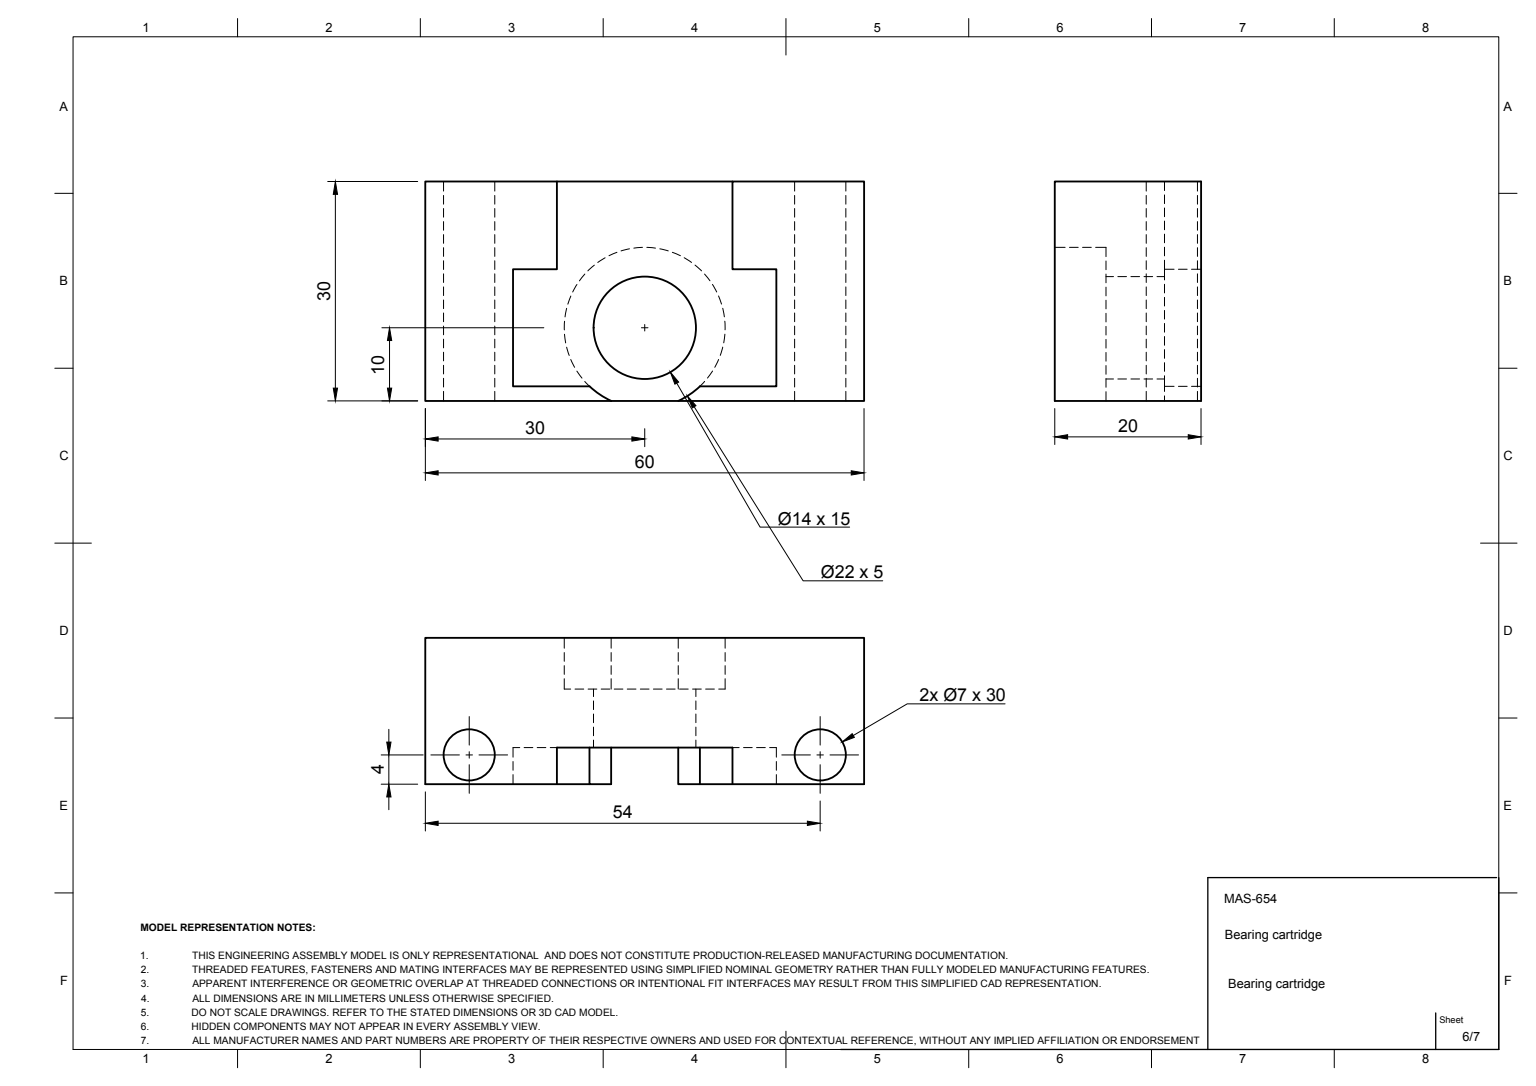
ISO-10303-21;
HEADER;
/* Generated by software containing ST-Developer
 * from STEP Tools, Inc. (www.steptools.com) 
 */

FILE_DESCRIPTION(
/* description */ ('Independent four-jaw lathe chuck,200mm body,40mm bore,36\X2\2013\X0\7
6mm nominal opposed jaw opening. Four shared machined T-jaws and model
ed partial M12x1.75 feed screws, native independent screw/slider links
, removable bolted bronze-bearing cartridges, fully captured ring/wash
er/head thrust stacks and registered bolted backplate. Custom spindle 
interface; no compatibility, speed, grip force or safety rating assign
ed.'),
/* implementation_level */ '2;1');

FILE_NAME(
/* name */ 'Bearing cartridge.step',
/* time_stamp */ '2026-11-09T20:24:54-08:00',
/* author */ (''),
/* organization */ (''),
/* preprocessor_version */ 'ST-DEVELOPER v20.2',
/* originating_system */ 'Autodesk Translation Framework v15.17.0.0',
/* authorisation */ '');

FILE_SCHEMA (('AUTOMOTIVE_DESIGN { 1 0 10303 214 3 1 1 }'));
ENDSEC;

DATA;
#10=MECHANICAL_DESIGN_GEOMETRIC_PRESENTATION_REPRESENTATION('',(#239),#69491);
#217=SHAPE_REPRESENTATION_RELATIONSHIP('SRR','None',#69574,#228);
#228=ADVANCED_BREP_SHAPE_REPRESENTATION('',(#250),#69483);
#239=STYLED_ITEM('',(#69638),#250);
#250=MANIFOLD_SOLID_BREP('Body1',#14734);
#345=FACE_BOUND('',#1827,.T.);
#346=FACE_BOUND('',#1832,.T.);
#347=FACE_BOUND('',#1835,.T.);
#348=FACE_BOUND('',#1836,.T.);
#349=FACE_BOUND('',#1849,.T.);
#350=FACE_BOUND('',#1850,.T.);
#462=PLANE('',#15459);
#463=PLANE('',#15461);
#464=PLANE('',#15462);
#465=PLANE('',#15463);
#466=PLANE('',#15464);
#467=PLANE('',#15469);
#468=PLANE('',#15471);
#469=PLANE('',#15472);
#470=PLANE('',#15473);
#471=PLANE('',#15474);
#472=PLANE('',#15475);
#473=PLANE('',#15476);
#474=PLANE('',#15477);
#475=PLANE('',#15478);
#476=PLANE('',#15479);
#477=PLANE('',#15480);
#478=PLANE('',#15481);
#994=FACE_OUTER_BOUND('',#1822,.T.);
#995=FACE_OUTER_BOUND('',#1823,.T.);
#996=FACE_OUTER_BOUND('',#1824,.T.);
#997=FACE_OUTER_BOUND('',#1825,.T.);
#998=FACE_OUTER_BOUND('',#1826,.T.);
#999=FACE_OUTER_BOUND('',#1828,.T.);
#1000=FACE_OUTER_BOUND('',#1829,.T.);
#1001=FACE_OUTER_BOUND('',#1830,.T.);
#1002=FACE_OUTER_BOUND('',#1831,.T.);
#1003=FACE_OUTER_BOUND('',#1833,.T.);
#1004=FACE_OUTER_BOUND('',#1834,.T.);
#1005=FACE_OUTER_BOUND('',#1837,.T.);
#1006=FACE_OUTER_BOUND('',#1838,.T.);
#1007=FACE_OUTER_BOUND('',#1839,.T.);
#1008=FACE_OUTER_BOUND('',#1840,.T.);
#1009=FACE_OUTER_BOUND('',#1841,.T.);
#1010=FACE_OUTER_BOUND('',#1842,.T.);
#1011=FACE_OUTER_BOUND('',#1843,.T.);
#1012=FACE_OUTER_BOUND('',#1844,.T.);
#1013=FACE_OUTER_BOUND('',#1845,.T.);
#1014=FACE_OUTER_BOUND('',#1846,.T.);
#1015=FACE_OUTER_BOUND('',#1847,.T.);
#1016=FACE_OUTER_BOUND('',#1848,.T.);
#1822=EDGE_LOOP('',(#11663,#11664,#11665,#11666));
#1823=EDGE_LOOP('',(#11667,#11668,#11669,#11670));
#1824=EDGE_LOOP('',(#11671,#11672,#11673,#11674));
#1825=EDGE_LOOP('',(#11675,#11676,#11677,#11678));
#1826=EDGE_LOOP('',(#11679,#11680,#11681,#11682,#11683,#11684,#11685,#11686,
#11687,#11688,#11689,#11690));
#1827=EDGE_LOOP('',(#11691));
#1828=EDGE_LOOP('',(#11692,#11693,#11694,#11695,#11696,#11697,#11698,#11699));
#1829=EDGE_LOOP('',(#11700,#11701,#11702,#11703,#11704,#11705,#11706,#11707));
#1830=EDGE_LOOP('',(#11708,#11709,#11710,#11711));
#1831=EDGE_LOOP('',(#11712,#11713));
#1832=EDGE_LOOP('',(#11714));
#1833=EDGE_LOOP('',(#11715,#11716,#11717,#11718));
#1834=EDGE_LOOP('',(#11719,#11720,#11721,#11722,#11723,#11724,#11725,#11726,
#11727,#11728,#11729,#11730));
#1835=EDGE_LOOP('',(#11731));
#1836=EDGE_LOOP('',(#11732));
#1837=EDGE_LOOP('',(#11733,#11734,#11735,#11736));
#1838=EDGE_LOOP('',(#11737,#11738,#11739,#11740));
#1839=EDGE_LOOP('',(#11741,#11742,#11743,#11744));
#1840=EDGE_LOOP('',(#11745,#11746,#11747,#11748));
#1841=EDGE_LOOP('',(#11749,#11750,#11751,#11752));
#1842=EDGE_LOOP('',(#11753,#11754,#11755,#11756));
#1843=EDGE_LOOP('',(#11757,#11758,#11759,#11760));
#1844=EDGE_LOOP('',(#11761,#11762,#11763,#11764));
#1845=EDGE_LOOP('',(#11765,#11766,#11767,#11768));
#1846=EDGE_LOOP('',(#11769,#11770,#11771,#11772,#11773,#11774));
#1847=EDGE_LOOP('',(#11775,#11776,#11777,#11778));
#1848=EDGE_LOOP('',(#11779,#11780,#11781,#11782,#11783,#11784,#11785,#11786));
#1849=EDGE_LOOP('',(#11787));
#1850=EDGE_LOOP('',(#11788));
#2291=CIRCLE('',#15448,3.5);
#2292=CIRCLE('',#15449,3.5);
#2293=CIRCLE('',#15451,3.5);
#2294=CIRCLE('',#15452,3.5);
#2295=CIRCLE('',#15454,11.);
#2296=CIRCLE('',#15455,11.);
#2297=CIRCLE('',#15457,11.);
#2298=CIRCLE('',#15458,11.);
#2299=CIRCLE('',#15460,7.);
#2300=CIRCLE('',#15465,11.);
#2301=CIRCLE('',#15466,7.);
#2302=CIRCLE('',#15468,11.);
#4032=LINE('',#50300,#4880);
#4033=LINE('',#50306,#4881);
#4034=LINE('',#50311,#4882);
#4035=LINE('',#50315,#4883);
#4036=LINE('',#50320,#4884);
#4037=LINE('',#50324,#4885);
#4038=LINE('',#50328,#4886);
#4039=LINE('',#50330,#4887);
#4040=LINE('',#50332,#4888);
#4041=LINE('',#50334,#4889);
#4042=LINE('',#50336,#4890);
#4043=LINE('',#50338,#4891);
#4044=LINE('',#50340,#4892);
#4045=LINE('',#50342,#4893);
#4046=LINE('',#50343,#4894);
#4047=LINE('',#50344,#4895);
#4048=LINE('',#50349,#4896);
#4049=LINE('',#50351,#4897);
#4050=LINE('',#50353,#4898);
#4051=LINE('',#50355,#4899);
#4052=LINE('',#50357,#4900);
#4053=LINE('',#50359,#4901);
#4054=LINE('',#50360,#4902);
#4055=LINE('',#50363,#4903);
#4056=LINE('',#50365,#4904);
#4057=LINE('',#50367,#4905);
#4058=LINE('',#50369,#4906);
#4059=LINE('',#50371,#4907);
#4060=LINE('',#50373,#4908);
#4061=LINE('',#50374,#4909);
#4062=LINE('',#50376,#4910);
#4063=LINE('',#50380,#4911);
#4064=LINE('',#50386,#4912);
#4065=LINE('',#50389,#4913);
#4066=LINE('',#50392,#4914);
#4067=LINE('',#50393,#4915);
#4068=LINE('',#50395,#4916);
#4069=LINE('',#50396,#4917);
#4070=LINE('',#50398,#4918);
#4071=LINE('',#50400,#4919);
#4072=LINE('',#50401,#4920);
#4073=LINE('',#50404,#4921);
#4074=LINE('',#50405,#4922);
#4075=LINE('',#50407,#4923);
#4076=LINE('',#50410,#4924);
#4077=LINE('',#50412,#4925);
#4078=LINE('',#50415,#4926);
#4079=LINE('',#50416,#4927);
#4080=LINE('',#50419,#4928);
#4081=LINE('',#50420,#4929);
#4082=LINE('',#50422,#4930);
#4880=VECTOR('',#17538,3.5);
#4881=VECTOR('',#17545,3.5);
#4882=VECTOR('',#17550,10.);
#4883=VECTOR('',#17553,10.);
#4884=VECTOR('',#17558,10.);
#4885=VECTOR('',#17561,10.);
#4886=VECTOR('',#17566,10.);
#4887=VECTOR('',#17567,10.);
#4888=VECTOR('',#17568,10.);
#4889=VECTOR('',#17569,10.);
#4890=VECTOR('',#17570,10.);
#4891=VECTOR('',#17571,10.);
#4892=VECTOR('',#17572,10.);
#4893=VECTOR('',#17573,10.);
#4894=VECTOR('',#17574,10.);
#4895=VECTOR('',#17575,10.);
#4896=VECTOR('',#17580,10.);
#4897=VECTOR('',#17581,10.);
#4898=VECTOR('',#17582,10.);
#4899=VECTOR('',#17583,10.);
#4900=VECTOR('',#17584,10.);
#4901=VECTOR('',#17585,10.);
#4902=VECTOR('',#17586,10.);
#4903=VECTOR('',#17589,10.);
#4904=VECTOR('',#17590,10.);
#4905=VECTOR('',#17591,10.);
#4906=VECTOR('',#17592,10.);
#4907=VECTOR('',#17593,10.);
#4908=VECTOR('',#17594,10.);
#4909=VECTOR('',#17595,10.);
#4910=VECTOR('',#17598,10.);
#4911=VECTOR('',#17601,10.);
#4912=VECTOR('',#17608,10.);
#4913=VECTOR('',#17611,10.);
#4914=VECTOR('',#17614,10.);
#4915=VECTOR('',#17615,10.);
#4916=VECTOR('',#17616,10.);
#4917=VECTOR('',#17617,10.);
#4918=VECTOR('',#17620,7.);
#4919=VECTOR('',#17623,10.);
#4920=VECTOR('',#17624,10.);
#4921=VECTOR('',#17629,10.);
#4922=VECTOR('',#17630,10.);
#4923=VECTOR('',#17633,10.);
#4924=VECTOR('',#17638,10.);
#4925=VECTOR('',#17641,10.);
#4926=VECTOR('',#17644,10.);
#4927=VECTOR('',#17645,10.);
#4928=VECTOR('',#17648,10.);
#4929=VECTOR('',#17649,10.);
#4930=VECTOR('',#17652,10.);
#6129=VERTEX_POINT('',#50297);
#6130=VERTEX_POINT('',#50299);
#6131=VERTEX_POINT('',#50303);
#6132=VERTEX_POINT('',#50305);
#6133=VERTEX_POINT('',#50309);
#6134=VERTEX_POINT('',#50310);
#6135=VERTEX_POINT('',#50312);
#6136=VERTEX_POINT('',#50314);
#6137=VERTEX_POINT('',#50318);
#6138=VERTEX_POINT('',#50319);
#6139=VERTEX_POINT('',#50321);
#6140=VERTEX_POINT('',#50323);
#6141=VERTEX_POINT('',#50327);
#6142=VERTEX_POINT('',#50329);
#6143=VERTEX_POINT('',#50331);
#6144=VERTEX_POINT('',#50333);
#6145=VERTEX_POINT('',#50335);
#6146=VERTEX_POINT('',#50337);
#6147=VERTEX_POINT('',#50339);
#6148=VERTEX_POINT('',#50341);
#6149=VERTEX_POINT('',#50345);
#6150=VERTEX_POINT('',#50348);
#6151=VERTEX_POINT('',#50350);
#6152=VERTEX_POINT('',#50352);
#6153=VERTEX_POINT('',#50354);
#6154=VERTEX_POINT('',#50356);
#6155=VERTEX_POINT('',#50358);
#6156=VERTEX_POINT('',#50362);
#6157=VERTEX_POINT('',#50364);
#6158=VERTEX_POINT('',#50366);
#6159=VERTEX_POINT('',#50368);
#6160=VERTEX_POINT('',#50370);
#6161=VERTEX_POINT('',#50372);
#6162=VERTEX_POINT('',#50378);
#6163=VERTEX_POINT('',#50379);
#6164=VERTEX_POINT('',#50382);
#6165=VERTEX_POINT('',#50385);
#6166=VERTEX_POINT('',#50387);
#6167=VERTEX_POINT('',#50391);
#6168=VERTEX_POINT('',#50394);
#6169=VERTEX_POINT('',#50414);
#6170=VERTEX_POINT('',#50418);
#8068=EDGE_CURVE('',#6129,#6129,#2291,.T.);
#8069=EDGE_CURVE('',#6129,#6130,#4032,.T.);
#8070=EDGE_CURVE('',#6130,#6130,#2292,.T.);
#8071=EDGE_CURVE('',#6131,#6131,#2293,.T.);
#8072=EDGE_CURVE('',#6131,#6132,#4033,.T.);
#8073=EDGE_CURVE('',#6132,#6132,#2294,.T.);
#8074=EDGE_CURVE('',#6133,#6134,#4034,.T.);
#8075=EDGE_CURVE('',#6135,#6133,#2295,.T.);
#8076=EDGE_CURVE('',#6136,#6135,#4035,.T.);
#8077=EDGE_CURVE('',#6136,#6134,#2296,.T.);
#8078=EDGE_CURVE('',#6137,#6138,#4036,.T.);
#8079=EDGE_CURVE('',#6137,#6139,#2297,.T.);
#8080=EDGE_CURVE('',#6140,#6139,#4037,.T.);
#8081=EDGE_CURVE('',#6138,#6140,#2298,.T.);
#8082=EDGE_CURVE('',#6136,#6141,#4038,.T.);
#8083=EDGE_CURVE('',#6142,#6141,#4039,.T.);
#8084=EDGE_CURVE('',#6142,#6143,#4040,.T.);
#8085=EDGE_CURVE('',#6144,#6143,#4041,.T.);
#8086=EDGE_CURVE('',#6145,#6144,#4042,.T.);
#8087=EDGE_CURVE('',#6145,#6146,#4043,.T.);
#8088=EDGE_CURVE('',#6146,#6147,#4044,.T.);
#8089=EDGE_CURVE('',#6147,#6148,#4045,.T.);
#8090=EDGE_CURVE('',#6148,#6139,#4046,.T.);
#8091=EDGE_CURVE('',#6134,#6137,#4047,.T.);
#8092=EDGE_CURVE('',#6149,#6149,#2299,.T.);
#8093=EDGE_CURVE('',#6133,#6150,#4048,.T.);
#8094=EDGE_CURVE('',#6150,#6151,#4049,.T.);
#8095=EDGE_CURVE('',#6152,#6151,#4050,.T.);
#8096=EDGE_CURVE('',#6152,#6153,#4051,.T.);
#8097=EDGE_CURVE('',#6153,#6154,#4052,.T.);
#8098=EDGE_CURVE('',#6154,#6155,#4053,.T.);
#8099=EDGE_CURVE('',#6155,#6135,#4054,.T.);
#8100=EDGE_CURVE('',#6140,#6156,#4055,.T.);
#8101=EDGE_CURVE('',#6156,#6157,#4056,.T.);
#8102=EDGE_CURVE('',#6157,#6158,#4057,.T.);
#8103=EDGE_CURVE('',#6158,#6159,#4058,.T.);
#8104=EDGE_CURVE('',#6160,#6159,#4059,.T.);
#8105=EDGE_CURVE('',#6161,#6160,#4060,.T.);
#8106=EDGE_CURVE('',#6161,#6138,#4061,.T.);
#8107=EDGE_CURVE('',#6141,#6155,#4062,.T.);
#8108=EDGE_CURVE('',#6162,#6163,#4063,.T.);
#8109=EDGE_CURVE('',#6163,#6162,#2300,.T.);
#8110=EDGE_CURVE('',#6164,#6164,#2301,.T.);
#8111=EDGE_CURVE('',#6165,#6162,#4064,.T.);
#8112=EDGE_CURVE('',#6166,#6165,#2302,.T.);
#8113=EDGE_CURVE('',#6163,#6166,#4065,.T.);
#8114=EDGE_CURVE('',#6167,#6161,#4066,.T.);
#8115=EDGE_CURVE('',#6165,#6167,#4067,.T.);
#8116=EDGE_CURVE('',#6168,#6166,#4068,.T.);
#8117=EDGE_CURVE('',#6150,#6168,#4069,.T.);
#8118=EDGE_CURVE('',#6164,#6149,#4070,.T.);
#8119=EDGE_CURVE('',#6143,#6153,#4071,.T.);
#8120=EDGE_CURVE('',#6154,#6142,#4072,.T.);
#8121=EDGE_CURVE('',#6147,#6157,#4073,.T.);
#8122=EDGE_CURVE('',#6156,#6148,#4074,.T.);
#8123=EDGE_CURVE('',#6158,#6146,#4075,.T.);
#8124=EDGE_CURVE('',#6144,#6152,#4076,.T.);
#8125=EDGE_CURVE('',#6159,#6145,#4077,.T.);
#8126=EDGE_CURVE('',#6169,#6160,#4078,.T.);
#8127=EDGE_CURVE('',#6167,#6169,#4079,.T.);
#8128=EDGE_CURVE('',#6170,#6169,#4080,.T.);
#8129=EDGE_CURVE('',#6168,#6170,#4081,.T.);
#8130=EDGE_CURVE('',#6151,#6170,#4082,.T.);
#11663=ORIENTED_EDGE('',*,*,#8068,.F.);
#11664=ORIENTED_EDGE('',*,*,#8069,.T.);
#11665=ORIENTED_EDGE('',*,*,#8070,.F.);
#11666=ORIENTED_EDGE('',*,*,#8069,.F.);
#11667=ORIENTED_EDGE('',*,*,#8071,.F.);
#11668=ORIENTED_EDGE('',*,*,#8072,.T.);
#11669=ORIENTED_EDGE('',*,*,#8073,.F.);
#11670=ORIENTED_EDGE('',*,*,#8072,.F.);
#11671=ORIENTED_EDGE('',*,*,#8074,.F.);
#11672=ORIENTED_EDGE('',*,*,#8075,.F.);
#11673=ORIENTED_EDGE('',*,*,#8076,.F.);
#11674=ORIENTED_EDGE('',*,*,#8077,.T.);
#11675=ORIENTED_EDGE('',*,*,#8078,.F.);
#11676=ORIENTED_EDGE('',*,*,#8079,.T.);
#11677=ORIENTED_EDGE('',*,*,#8080,.F.);
#11678=ORIENTED_EDGE('',*,*,#8081,.F.);
#11679=ORIENTED_EDGE('',*,*,#8082,.T.);
#11680=ORIENTED_EDGE('',*,*,#8083,.F.);
#11681=ORIENTED_EDGE('',*,*,#8084,.T.);
#11682=ORIENTED_EDGE('',*,*,#8085,.F.);
#11683=ORIENTED_EDGE('',*,*,#8086,.F.);
#11684=ORIENTED_EDGE('',*,*,#8087,.T.);
#11685=ORIENTED_EDGE('',*,*,#8088,.T.);
#11686=ORIENTED_EDGE('',*,*,#8089,.T.);
#11687=ORIENTED_EDGE('',*,*,#8090,.T.);
#11688=ORIENTED_EDGE('',*,*,#8079,.F.);
#11689=ORIENTED_EDGE('',*,*,#8091,.F.);
#11690=ORIENTED_EDGE('',*,*,#8077,.F.);
#11691=ORIENTED_EDGE('',*,*,#8092,.T.);
#11692=ORIENTED_EDGE('',*,*,#8075,.T.);
#11693=ORIENTED_EDGE('',*,*,#8093,.T.);
#11694=ORIENTED_EDGE('',*,*,#8094,.T.);
#11695=ORIENTED_EDGE('',*,*,#8095,.F.);
#11696=ORIENTED_EDGE('',*,*,#8096,.T.);
#11697=ORIENTED_EDGE('',*,*,#8097,.T.);
#11698=ORIENTED_EDGE('',*,*,#8098,.T.);
#11699=ORIENTED_EDGE('',*,*,#8099,.T.);
#11700=ORIENTED_EDGE('',*,*,#8081,.T.);
#11701=ORIENTED_EDGE('',*,*,#8100,.T.);
#11702=ORIENTED_EDGE('',*,*,#8101,.T.);
#11703=ORIENTED_EDGE('',*,*,#8102,.T.);
#11704=ORIENTED_EDGE('',*,*,#8103,.T.);
#11705=ORIENTED_EDGE('',*,*,#8104,.F.);
#11706=ORIENTED_EDGE('',*,*,#8105,.F.);
#11707=ORIENTED_EDGE('',*,*,#8106,.T.);
#11708=ORIENTED_EDGE('',*,*,#8076,.T.);
#11709=ORIENTED_EDGE('',*,*,#8099,.F.);
#11710=ORIENTED_EDGE('',*,*,#8107,.F.);
#11711=ORIENTED_EDGE('',*,*,#8082,.F.);
#11712=ORIENTED_EDGE('',*,*,#8108,.F.);
#11713=ORIENTED_EDGE('',*,*,#8109,.F.);
#11714=ORIENTED_EDGE('',*,*,#8110,.F.);
#11715=ORIENTED_EDGE('',*,*,#8111,.F.);
#11716=ORIENTED_EDGE('',*,*,#8112,.F.);
#11717=ORIENTED_EDGE('',*,*,#8113,.F.);
#11718=ORIENTED_EDGE('',*,*,#8109,.T.);
#11719=ORIENTED_EDGE('',*,*,#8078,.T.);
#11720=ORIENTED_EDGE('',*,*,#8106,.F.);
#11721=ORIENTED_EDGE('',*,*,#8114,.F.);
#11722=ORIENTED_EDGE('',*,*,#8115,.F.);
#11723=ORIENTED_EDGE('',*,*,#8111,.T.);
#11724=ORIENTED_EDGE('',*,*,#8108,.T.);
#11725=ORIENTED_EDGE('',*,*,#8113,.T.);
#11726=ORIENTED_EDGE('',*,*,#8116,.F.);
#11727=ORIENTED_EDGE('',*,*,#8117,.F.);
#11728=ORIENTED_EDGE('',*,*,#8093,.F.);
#11729=ORIENTED_EDGE('',*,*,#8074,.T.);
#11730=ORIENTED_EDGE('',*,*,#8091,.T.);
#11731=ORIENTED_EDGE('',*,*,#8070,.T.);
#11732=ORIENTED_EDGE('',*,*,#8073,.T.);
#11733=ORIENTED_EDGE('',*,*,#8110,.T.);
#11734=ORIENTED_EDGE('',*,*,#8118,.T.);
#11735=ORIENTED_EDGE('',*,*,#8092,.F.);
#11736=ORIENTED_EDGE('',*,*,#8118,.F.);
#11737=ORIENTED_EDGE('',*,*,#8119,.F.);
#11738=ORIENTED_EDGE('',*,*,#8084,.F.);
#11739=ORIENTED_EDGE('',*,*,#8120,.F.);
#11740=ORIENTED_EDGE('',*,*,#8097,.F.);
#11741=ORIENTED_EDGE('',*,*,#8120,.T.);
#11742=ORIENTED_EDGE('',*,*,#8083,.T.);
#11743=ORIENTED_EDGE('',*,*,#8107,.T.);
#11744=ORIENTED_EDGE('',*,*,#8098,.F.);
#11745=ORIENTED_EDGE('',*,*,#8121,.T.);
#11746=ORIENTED_EDGE('',*,*,#8101,.F.);
#11747=ORIENTED_EDGE('',*,*,#8122,.T.);
#11748=ORIENTED_EDGE('',*,*,#8089,.F.);
#11749=ORIENTED_EDGE('',*,*,#8123,.F.);
#11750=ORIENTED_EDGE('',*,*,#8102,.F.);
#11751=ORIENTED_EDGE('',*,*,#8121,.F.);
#11752=ORIENTED_EDGE('',*,*,#8088,.F.);
#11753=ORIENTED_EDGE('',*,*,#8080,.T.);
#11754=ORIENTED_EDGE('',*,*,#8090,.F.);
#11755=ORIENTED_EDGE('',*,*,#8122,.F.);
#11756=ORIENTED_EDGE('',*,*,#8100,.F.);
#11757=ORIENTED_EDGE('',*,*,#8124,.F.);
#11758=ORIENTED_EDGE('',*,*,#8085,.T.);
#11759=ORIENTED_EDGE('',*,*,#8119,.T.);
#11760=ORIENTED_EDGE('',*,*,#8096,.F.);
#11761=ORIENTED_EDGE('',*,*,#8125,.F.);
#11762=ORIENTED_EDGE('',*,*,#8103,.F.);
#11763=ORIENTED_EDGE('',*,*,#8123,.T.);
#11764=ORIENTED_EDGE('',*,*,#8087,.F.);
#11765=ORIENTED_EDGE('',*,*,#8114,.T.);
#11766=ORIENTED_EDGE('',*,*,#8105,.T.);
#11767=ORIENTED_EDGE('',*,*,#8126,.F.);
#11768=ORIENTED_EDGE('',*,*,#8127,.F.);
#11769=ORIENTED_EDGE('',*,*,#8112,.T.);
#11770=ORIENTED_EDGE('',*,*,#8115,.T.);
#11771=ORIENTED_EDGE('',*,*,#8127,.T.);
#11772=ORIENTED_EDGE('',*,*,#8128,.F.);
#11773=ORIENTED_EDGE('',*,*,#8129,.F.);
#11774=ORIENTED_EDGE('',*,*,#8116,.T.);
#11775=ORIENTED_EDGE('',*,*,#8117,.T.);
#11776=ORIENTED_EDGE('',*,*,#8129,.T.);
#11777=ORIENTED_EDGE('',*,*,#8130,.F.);
#11778=ORIENTED_EDGE('',*,*,#8094,.F.);
#11779=ORIENTED_EDGE('',*,*,#8124,.T.);
#11780=ORIENTED_EDGE('',*,*,#8095,.T.);
#11781=ORIENTED_EDGE('',*,*,#8130,.T.);
#11782=ORIENTED_EDGE('',*,*,#8128,.T.);
#11783=ORIENTED_EDGE('',*,*,#8126,.T.);
#11784=ORIENTED_EDGE('',*,*,#8104,.T.);
#11785=ORIENTED_EDGE('',*,*,#8125,.T.);
#11786=ORIENTED_EDGE('',*,*,#8086,.T.);
#11787=ORIENTED_EDGE('',*,*,#8068,.T.);
#11788=ORIENTED_EDGE('',*,*,#8071,.T.);
#13710=CYLINDRICAL_SURFACE('',#15447,3.5);
#13711=CYLINDRICAL_SURFACE('',#15450,3.5);
#13712=CYLINDRICAL_SURFACE('',#15453,11.);
#13713=CYLINDRICAL_SURFACE('',#15456,11.);
#13714=CYLINDRICAL_SURFACE('',#15467,11.);
#13715=CYLINDRICAL_SURFACE('',#15470,7.);
#14422=ADVANCED_FACE('',(#994),#13710,.F.);
#14423=ADVANCED_FACE('',(#995),#13711,.F.);
#14424=ADVANCED_FACE('',(#996),#13712,.F.);
#14425=ADVANCED_FACE('',(#997),#13713,.F.);
#14426=ADVANCED_FACE('',(#998,#345),#462,.F.);
#14427=ADVANCED_FACE('',(#999),#463,.T.);
#14428=ADVANCED_FACE('',(#1000),#464,.T.);
#14429=ADVANCED_FACE('',(#1001),#465,.F.);
#14430=ADVANCED_FACE('',(#1002,#346),#466,.F.);
#14431=ADVANCED_FACE('',(#1003),#13714,.F.);
#14432=ADVANCED_FACE('',(#1004,#347,#348),#467,.F.);
#14433=ADVANCED_FACE('',(#1005),#13715,.F.);
#14434=ADVANCED_FACE('',(#1006),#468,.F.);
#14435=ADVANCED_FACE('',(#1007),#469,.F.);
#14436=ADVANCED_FACE('',(#1008),#470,.F.);
#14437=ADVANCED_FACE('',(#1009),#471,.F.);
#14438=ADVANCED_FACE('',(#1010),#472,.F.);
#14439=ADVANCED_FACE('',(#1011),#473,.F.);
#14440=ADVANCED_FACE('',(#1012),#474,.F.);
#14441=ADVANCED_FACE('',(#1013),#475,.T.);
#14442=ADVANCED_FACE('',(#1014),#476,.T.);
#14443=ADVANCED_FACE('',(#1015),#477,.T.);
#14444=ADVANCED_FACE('',(#1016,#349,#350),#478,.T.);
#14734=CLOSED_SHELL('',(#14422,#14423,#14424,#14425,#14426,#14427,#14428,
#14429,#14430,#14431,#14432,#14433,#14434,#14435,#14436,#14437,#14438,#14439,
#14440,#14441,#14442,#14443,#14444));
#15446=AXIS2_PLACEMENT_3D('',#50295,#17532,#17533);
#15447=AXIS2_PLACEMENT_3D('',#50296,#17534,#17535);
#15448=AXIS2_PLACEMENT_3D('',#50298,#17536,#17537);
#15449=AXIS2_PLACEMENT_3D('',#50301,#17539,#17540);
#15450=AXIS2_PLACEMENT_3D('',#50302,#17541,#17542);
#15451=AXIS2_PLACEMENT_3D('',#50304,#17543,#17544);
#15452=AXIS2_PLACEMENT_3D('',#50307,#17546,#17547);
#15453=AXIS2_PLACEMENT_3D('',#50308,#17548,#17549);
#15454=AXIS2_PLACEMENT_3D('',#50313,#17551,#17552);
#15455=AXIS2_PLACEMENT_3D('',#50316,#17554,#17555);
#15456=AXIS2_PLACEMENT_3D('',#50317,#17556,#17557);
#15457=AXIS2_PLACEMENT_3D('',#50322,#17559,#17560);
#15458=AXIS2_PLACEMENT_3D('',#50325,#17562,#17563);
#15459=AXIS2_PLACEMENT_3D('',#50326,#17564,#17565);
#15460=AXIS2_PLACEMENT_3D('',#50346,#17576,#17577);
#15461=AXIS2_PLACEMENT_3D('',#50347,#17578,#17579);
#15462=AXIS2_PLACEMENT_3D('',#50361,#17587,#17588);
#15463=AXIS2_PLACEMENT_3D('',#50375,#17596,#17597);
#15464=AXIS2_PLACEMENT_3D('',#50377,#17599,#17600);
#15465=AXIS2_PLACEMENT_3D('',#50381,#17602,#17603);
#15466=AXIS2_PLACEMENT_3D('',#50383,#17604,#17605);
#15467=AXIS2_PLACEMENT_3D('',#50384,#17606,#17607);
#15468=AXIS2_PLACEMENT_3D('',#50388,#17609,#17610);
#15469=AXIS2_PLACEMENT_3D('',#50390,#17612,#17613);
#15470=AXIS2_PLACEMENT_3D('',#50397,#17618,#17619);
#15471=AXIS2_PLACEMENT_3D('',#50399,#17621,#17622);
#15472=AXIS2_PLACEMENT_3D('',#50402,#17625,#17626);
#15473=AXIS2_PLACEMENT_3D('',#50403,#17627,#17628);
#15474=AXIS2_PLACEMENT_3D('',#50406,#17631,#17632);
#15475=AXIS2_PLACEMENT_3D('',#50408,#17634,#17635);
#15476=AXIS2_PLACEMENT_3D('',#50409,#17636,#17637);
#15477=AXIS2_PLACEMENT_3D('',#50411,#17639,#17640);
#15478=AXIS2_PLACEMENT_3D('',#50413,#17642,#17643);
#15479=AXIS2_PLACEMENT_3D('',#50417,#17646,#17647);
#15480=AXIS2_PLACEMENT_3D('',#50421,#17650,#17651);
#15481=AXIS2_PLACEMENT_3D('',#50423,#17653,#17654);
#17532=DIRECTION('axis',(0.,0.,1.));
#17533=DIRECTION('refdir',(1.,0.,0.));
#17534=DIRECTION('center_axis',(0.,0.,-1.));
#17535=DIRECTION('ref_axis',(1.,0.,0.));
#17536=DIRECTION('center_axis',(0.,0.,-1.));
#17537=DIRECTION('ref_axis',(1.,0.,0.));
#17538=DIRECTION('',(0.,0.,-1.));
#17539=DIRECTION('center_axis',(0.,0.,1.));
#17540=DIRECTION('ref_axis',(1.,0.,0.));
#17541=DIRECTION('center_axis',(0.,0.,-1.));
#17542=DIRECTION('ref_axis',(1.,0.,0.));
#17543=DIRECTION('center_axis',(0.,0.,-1.));
#17544=DIRECTION('ref_axis',(1.,0.,0.));
#17545=DIRECTION('',(0.,0.,-1.));
#17546=DIRECTION('center_axis',(0.,0.,1.));
#17547=DIRECTION('ref_axis',(1.,0.,0.));
#17548=DIRECTION('center_axis',(1.,0.,0.));
#17549=DIRECTION('ref_axis',(0.,-1.,0.));
#17550=DIRECTION('',(1.,0.,0.));
#17551=DIRECTION('center_axis',(1.,0.,0.));
#17552=DIRECTION('ref_axis',(0.,-1.,0.));
#17553=DIRECTION('',(-1.,0.,0.));
#17554=DIRECTION('center_axis',(1.,0.,0.));
#17555=DIRECTION('ref_axis',(0.,-1.,0.));
#17556=DIRECTION('center_axis',(1.,0.,0.));
#17557=DIRECTION('ref_axis',(0.,-1.,0.));
#17558=DIRECTION('',(-1.,0.,0.));
#17559=DIRECTION('center_axis',(1.,0.,0.));
#17560=DIRECTION('ref_axis',(0.,-1.,0.));
#17561=DIRECTION('',(1.,0.,0.));
#17562=DIRECTION('center_axis',(1.,0.,0.));
#17563=DIRECTION('ref_axis',(0.,-1.,0.));
#17564=DIRECTION('center_axis',(1.,0.,0.));
#17565=DIRECTION('ref_axis',(0.,-1.,0.));
#17566=DIRECTION('',(0.,-1.,0.));
#17567=DIRECTION('',(0.,0.,-1.));
#17568=DIRECTION('',(0.,1.,0.));
#17569=DIRECTION('',(0.,0.,-1.));
#17570=DIRECTION('',(0.,-1.,0.));
#17571=DIRECTION('',(0.,0.,-1.));
#17572=DIRECTION('',(0.,1.,0.));
#17573=DIRECTION('',(0.,0.,-1.));
#17574=DIRECTION('',(0.,-1.,0.));
#17575=DIRECTION('',(0.,1.,0.));
#17576=DIRECTION('center_axis',(1.,0.,0.));
#17577=DIRECTION('ref_axis',(0.,1.,0.));
#17578=DIRECTION('center_axis',(-1.,0.,0.));
#17579=DIRECTION('ref_axis',(0.,-1.,0.));
#17580=DIRECTION('',(0.,-1.,0.));
#17581=DIRECTION('',(0.,0.,1.));
#17582=DIRECTION('',(0.,-1.,0.));
#17583=DIRECTION('',(0.,0.,-1.));
#17584=DIRECTION('',(0.,-1.,0.));
#17585=DIRECTION('',(0.,0.,-1.));
#17586=DIRECTION('',(0.,1.,0.));
#17587=DIRECTION('center_axis',(-1.,0.,0.));
#17588=DIRECTION('ref_axis',(0.,-1.,0.));
#17589=DIRECTION('',(0.,1.,0.));
#17590=DIRECTION('',(0.,0.,1.));
#17591=DIRECTION('',(0.,-1.,0.));
#17592=DIRECTION('',(0.,0.,1.));
#17593=DIRECTION('',(0.,-1.,0.));
#17594=DIRECTION('',(0.,0.,1.));
#17595=DIRECTION('',(0.,-1.,0.));
#17596=DIRECTION('center_axis',(0.,0.,-1.));
#17597=DIRECTION('ref_axis',(-1.,0.,0.));
#17598=DIRECTION('',(-1.,0.,0.));
#17599=DIRECTION('center_axis',(-1.,0.,0.));
#17600=DIRECTION('ref_axis',(0.,1.,0.));
#17601=DIRECTION('',(0.,-1.,0.));
#17602=DIRECTION('center_axis',(-1.,0.,0.));
#17603=DIRECTION('ref_axis',(0.,1.,0.));
#17604=DIRECTION('center_axis',(1.,0.,0.));
#17605=DIRECTION('ref_axis',(0.,1.,0.));
#17606=DIRECTION('center_axis',(-1.,0.,0.));
#17607=DIRECTION('ref_axis',(0.,6.12323399573677E-17,1.));
#17608=DIRECTION('',(-1.,0.,0.));
#17609=DIRECTION('center_axis',(-1.,0.,0.));
#17610=DIRECTION('ref_axis',(0.,1.,0.));
#17611=DIRECTION('',(1.,0.,0.));
#17612=DIRECTION('center_axis',(0.,0.,1.));
#17613=DIRECTION('ref_axis',(1.,0.,0.));
#17614=DIRECTION('',(-1.,0.,0.));
#17615=DIRECTION('',(0.,1.,0.));
#17616=DIRECTION('',(0.,1.,0.));
#17617=DIRECTION('',(1.,0.,0.));
#17618=DIRECTION('center_axis',(-1.,0.,0.));
#17619=DIRECTION('ref_axis',(0.,1.,0.));
#17620=DIRECTION('',(-1.,0.,0.));
#17621=DIRECTION('center_axis',(0.,0.,1.));
#17622=DIRECTION('ref_axis',(1.,0.,0.));
#17623=DIRECTION('',(-1.,0.,0.));
#17624=DIRECTION('',(1.,0.,0.));
#17625=DIRECTION('center_axis',(0.,-1.,0.));
#17626=DIRECTION('ref_axis',(-1.,0.,0.));
#17627=DIRECTION('center_axis',(0.,1.,0.));
#17628=DIRECTION('ref_axis',(1.,0.,0.));
#17629=DIRECTION('',(-1.,0.,0.));
#17630=DIRECTION('',(1.,0.,0.));
#17631=DIRECTION('center_axis',(0.,0.,1.));
#17632=DIRECTION('ref_axis',(1.,0.,0.));
#17633=DIRECTION('',(1.,0.,0.));
#17634=DIRECTION('center_axis',(0.,0.,-1.));
#17635=DIRECTION('ref_axis',(-1.,0.,0.));
#17636=DIRECTION('center_axis',(0.,-1.,0.));
#17637=DIRECTION('ref_axis',(-1.,0.,0.));
#17638=DIRECTION('',(-1.,0.,0.));
#17639=DIRECTION('center_axis',(0.,1.,0.));
#17640=DIRECTION('ref_axis',(1.,0.,0.));
#17641=DIRECTION('',(1.,0.,0.));
#17642=DIRECTION('center_axis',(0.,1.,0.));
#17643=DIRECTION('ref_axis',(-1.,0.,0.));
#17644=DIRECTION('',(-1.,0.,0.));
#17645=DIRECTION('',(0.,0.,1.));
#17646=DIRECTION('center_axis',(1.,0.,0.));
#17647=DIRECTION('ref_axis',(0.,1.,0.));
#17648=DIRECTION('',(0.,1.,0.));
#17649=DIRECTION('',(0.,0.,1.));
#17650=DIRECTION('center_axis',(0.,-1.,0.));
#17651=DIRECTION('ref_axis',(1.,0.,0.));
#17652=DIRECTION('',(1.,0.,0.));
#17653=DIRECTION('center_axis',(0.,0.,1.));
#17654=DIRECTION('ref_axis',(1.,0.,0.));
#50295=CARTESIAN_POINT('',(0.,0.,0.));
#50296=CARTESIAN_POINT('Origin',(92.,-24.,25.));
#50297=CARTESIAN_POINT('',(88.5,-24.,40.));
#50298=CARTESIAN_POINT('Origin',(92.,-24.,40.));
#50299=CARTESIAN_POINT('',(88.5,-24.,10.));
#50300=CARTESIAN_POINT('',(88.5,-24.,25.));
#50301=CARTESIAN_POINT('Origin',(92.,-24.,10.));
#50302=CARTESIAN_POINT('Origin',(92.,24.,25.));
#50303=CARTESIAN_POINT('',(88.5,24.,40.));
#50304=CARTESIAN_POINT('Origin',(92.,24.,40.));
#50305=CARTESIAN_POINT('',(88.5,24.,10.));
#50306=CARTESIAN_POINT('',(88.5,24.,25.));
#50307=CARTESIAN_POINT('Origin',(92.,24.,10.));
#50308=CARTESIAN_POINT('Origin',(90.5,0.,20.));
#50309=CARTESIAN_POINT('',(88.,-4.58257569495584,10.));
#50310=CARTESIAN_POINT('',(93.,-4.58257569495584,10.));
#50311=CARTESIAN_POINT('',(90.5,-4.58257569495584,10.));
#50312=CARTESIAN_POINT('',(88.,-7.54983443527075,12.));
#50313=CARTESIAN_POINT('Origin',(88.,0.,20.));
#50314=CARTESIAN_POINT('',(93.,-7.54983443527075,12.));
#50315=CARTESIAN_POINT('',(90.5,-7.54983443527075,12.));
#50316=CARTESIAN_POINT('Origin',(93.,0.,20.));
#50317=CARTESIAN_POINT('Origin',(90.5,0.,20.));
#50318=CARTESIAN_POINT('',(93.,4.58257569495584,10.));
#50319=CARTESIAN_POINT('',(88.,4.58257569495584,10.));
#50320=CARTESIAN_POINT('',(90.5,4.58257569495584,10.));
#50321=CARTESIAN_POINT('',(93.,7.54983443527075,12.));
#50322=CARTESIAN_POINT('Origin',(93.,0.,20.));
#50323=CARTESIAN_POINT('',(88.,7.54983443527075,12.));
#50324=CARTESIAN_POINT('',(90.5,7.54983443527075,12.));
#50325=CARTESIAN_POINT('Origin',(88.,0.,20.));
#50326=CARTESIAN_POINT('Origin',(93.,12.,40.));
#50327=CARTESIAN_POINT('',(93.,-18.,12.));
#50328=CARTESIAN_POINT('',(93.,-18.,12.));
#50329=CARTESIAN_POINT('',(93.,-18.,28.));
#50330=CARTESIAN_POINT('',(93.,-18.,28.));
#50331=CARTESIAN_POINT('',(93.,-12.,28.));
#50332=CARTESIAN_POINT('',(93.,-18.,28.));
#50333=CARTESIAN_POINT('',(93.,-12.,40.));
#50334=CARTESIAN_POINT('',(93.,-12.,40.));
#50335=CARTESIAN_POINT('',(93.,12.,40.));
#50336=CARTESIAN_POINT('',(93.,6.,40.));
#50337=CARTESIAN_POINT('',(93.,12.,28.));
#50338=CARTESIAN_POINT('',(93.,12.,40.));
#50339=CARTESIAN_POINT('',(93.,18.,28.));
#50340=CARTESIAN_POINT('',(93.,-18.,28.));
#50341=CARTESIAN_POINT('',(93.,18.,12.));
#50342=CARTESIAN_POINT('',(93.,18.,28.));
#50343=CARTESIAN_POINT('',(93.,-18.,12.));
#50344=CARTESIAN_POINT('',(93.,0.,10.));
#50345=CARTESIAN_POINT('',(93.,-7.,20.));
#50346=CARTESIAN_POINT('Origin',(93.,0.,20.));
#50347=CARTESIAN_POINT('Origin',(88.,30.,10.));
#50348=CARTESIAN_POINT('',(88.,-30.,10.));
#50349=CARTESIAN_POINT('',(88.,30.,10.));
#50350=CARTESIAN_POINT('',(88.,-30.,40.));
#50351=CARTESIAN_POINT('',(88.,-30.,10.));
#50352=CARTESIAN_POINT('',(88.,-12.,40.));
#50353=CARTESIAN_POINT('',(88.,30.,40.));
#50354=CARTESIAN_POINT('',(88.,-12.,28.));
#50355=CARTESIAN_POINT('',(88.,-12.,25.));
#50356=CARTESIAN_POINT('',(88.,-18.,28.));
#50357=CARTESIAN_POINT('',(88.,15.,28.));
#50358=CARTESIAN_POINT('',(88.,-18.,12.));
#50359=CARTESIAN_POINT('',(88.,-18.,19.));
#50360=CARTESIAN_POINT('',(88.,15.,12.));
#50361=CARTESIAN_POINT('Origin',(88.,30.,10.));
#50362=CARTESIAN_POINT('',(88.,18.,12.));
#50363=CARTESIAN_POINT('',(88.,15.,12.));
#50364=CARTESIAN_POINT('',(88.,18.,28.));
#50365=CARTESIAN_POINT('',(88.,18.,19.));
#50366=CARTESIAN_POINT('',(88.,12.,28.));
#50367=CARTESIAN_POINT('',(88.,15.,28.));
#50368=CARTESIAN_POINT('',(88.,12.,40.));
#50369=CARTESIAN_POINT('',(88.,12.,25.));
#50370=CARTESIAN_POINT('',(88.,30.,40.));
#50371=CARTESIAN_POINT('',(88.,30.,40.));
#50372=CARTESIAN_POINT('',(88.,30.,10.));
#50373=CARTESIAN_POINT('',(88.,30.,10.));
#50374=CARTESIAN_POINT('',(88.,30.,10.));
#50375=CARTESIAN_POINT('Origin',(90.5,0.,12.));
#50376=CARTESIAN_POINT('',(88.,-18.,12.));
#50377=CARTESIAN_POINT('Origin',(101.,0.,20.));
#50378=CARTESIAN_POINT('',(101.,4.58257569495584,10.));
#50379=CARTESIAN_POINT('',(101.,-4.58257569495584,10.));
#50380=CARTESIAN_POINT('',(101.,0.,10.));
#50381=CARTESIAN_POINT('Origin',(101.,0.,20.));
#50382=CARTESIAN_POINT('',(101.,-7.,20.));
#50383=CARTESIAN_POINT('Origin',(101.,0.,20.));
#50384=CARTESIAN_POINT('Origin',(104.5,0.,20.));
#50385=CARTESIAN_POINT('',(108.,4.58257569495584,10.));
#50386=CARTESIAN_POINT('',(104.5,4.58257569495584,10.));
#50387=CARTESIAN_POINT('',(108.,-4.58257569495584,10.));
#50388=CARTESIAN_POINT('Origin',(108.,0.,20.));
#50389=CARTESIAN_POINT('',(104.5,-4.58257569495584,10.));
#50390=CARTESIAN_POINT('Origin',(98.,0.,10.));
#50391=CARTESIAN_POINT('',(108.,30.,10.));
#50392=CARTESIAN_POINT('',(108.,30.,10.));
#50393=CARTESIAN_POINT('',(108.,-30.,10.));
#50394=CARTESIAN_POINT('',(108.,-30.,10.));
#50395=CARTESIAN_POINT('',(108.,-30.,10.));
#50396=CARTESIAN_POINT('',(88.,-30.,10.));
#50397=CARTESIAN_POINT('Origin',(100.5,0.,20.));
#50398=CARTESIAN_POINT('',(100.5,-7.,20.));
#50399=CARTESIAN_POINT('Origin',(90.5,0.,28.));
#50400=CARTESIAN_POINT('',(88.,-12.,28.));
#50401=CARTESIAN_POINT('',(88.,-18.,28.));
#50402=CARTESIAN_POINT('Origin',(93.,-18.,28.));
#50403=CARTESIAN_POINT('Origin',(88.,18.,28.));
#50404=CARTESIAN_POINT('',(93.,18.,28.));
#50405=CARTESIAN_POINT('',(93.,18.,12.));
#50406=CARTESIAN_POINT('Origin',(90.5,0.,28.));
#50407=CARTESIAN_POINT('',(93.,12.,28.));
#50408=CARTESIAN_POINT('Origin',(90.5,0.,12.));
#50409=CARTESIAN_POINT('Origin',(93.,-12.,40.));
#50410=CARTESIAN_POINT('',(95.5,-12.,40.));
#50411=CARTESIAN_POINT('Origin',(88.,12.,40.));
#50412=CARTESIAN_POINT('',(93.,12.,40.));
#50413=CARTESIAN_POINT('Origin',(108.,30.,10.));
#50414=CARTESIAN_POINT('',(108.,30.,40.));
#50415=CARTESIAN_POINT('',(108.,30.,40.));
#50416=CARTESIAN_POINT('',(108.,30.,10.));
#50417=CARTESIAN_POINT('Origin',(108.,-30.,10.));
#50418=CARTESIAN_POINT('',(108.,-30.,40.));
#50419=CARTESIAN_POINT('',(108.,-30.,40.));
#50420=CARTESIAN_POINT('',(108.,-30.,10.));
#50421=CARTESIAN_POINT('Origin',(88.,-30.,10.));
#50422=CARTESIAN_POINT('',(88.,-30.,40.));
#50423=CARTESIAN_POINT('Origin',(98.,0.,40.));
#69470=UNCERTAINTY_MEASURE_WITH_UNIT(LENGTH_MEASURE(0.01),#69492,
'DISTANCE_ACCURACY_VALUE',
'Maximum model space distance between geometric entities at asserted c
onnectivities');
#69478=UNCERTAINTY_MEASURE_WITH_UNIT(LENGTH_MEASURE(0.01),#69492,
'DISTANCE_ACCURACY_VALUE',
'Maximum model space distance between geometric entities at asserted c
onnectivities');
#69483=(
GEOMETRIC_REPRESENTATION_CONTEXT(3)
GLOBAL_UNCERTAINTY_ASSIGNED_CONTEXT((#69470))
GLOBAL_UNIT_ASSIGNED_CONTEXT((#69492,#69494,#69495))
REPRESENTATION_CONTEXT('','3D')
);
#69491=(
GEOMETRIC_REPRESENTATION_CONTEXT(3)
GLOBAL_UNCERTAINTY_ASSIGNED_CONTEXT((#69478))
GLOBAL_UNIT_ASSIGNED_CONTEXT((#69492,#69494,#69495))
REPRESENTATION_CONTEXT('','3D')
);
#69492=(
LENGTH_UNIT()
NAMED_UNIT(*)
SI_UNIT(.MILLI.,.METRE.)
);
#69494=(
NAMED_UNIT(*)
PLANE_ANGLE_UNIT()
SI_UNIT($,.RADIAN.)
);
#69495=(
NAMED_UNIT(*)
SI_UNIT($,.STERADIAN.)
SOLID_ANGLE_UNIT()
);
#69500=SHAPE_DEFINITION_REPRESENTATION(#69512,#69574);
#69512=PRODUCT_DEFINITION_SHAPE('',$,#69587);
#69574=SHAPE_REPRESENTATION('',(#15446),#69483);
#69582=PRODUCT_DEFINITION_CONTEXT('part definition',#69620,'design');
#69587=PRODUCT_DEFINITION('Bearing cartridge','Bearing cartridge',#69599,
#69582);
#69599=PRODUCT_DEFINITION_FORMATION('',$,#69626);
#69620=APPLICATION_CONTEXT(
'Core Data for Automotive Mechanical Design Process');
#69621=PRODUCT_CONTEXT('part definition',#69620,'mechanical');
#69626=PRODUCT('Bearing cartridge','Bearing cartridge',$,(#69621));
#69638=PRESENTATION_STYLE_ASSIGNMENT((#69648));
#69648=SURFACE_STYLE_USAGE(.BOTH.,#69658);
#69658=SURFACE_SIDE_STYLE('',(#69668));
#69668=SURFACE_STYLE_FILL_AREA(#69678);
#69678=FILL_AREA_STYLE('Light blue',(#69688));
#69688=FILL_AREA_STYLE_COLOUR('Light blue',#69698);
#69698=COLOUR_RGB('Light blue',0.662745098039216,0.831372549019608,0.949019607843137);
ENDSEC;
END-ISO-10303-21;
